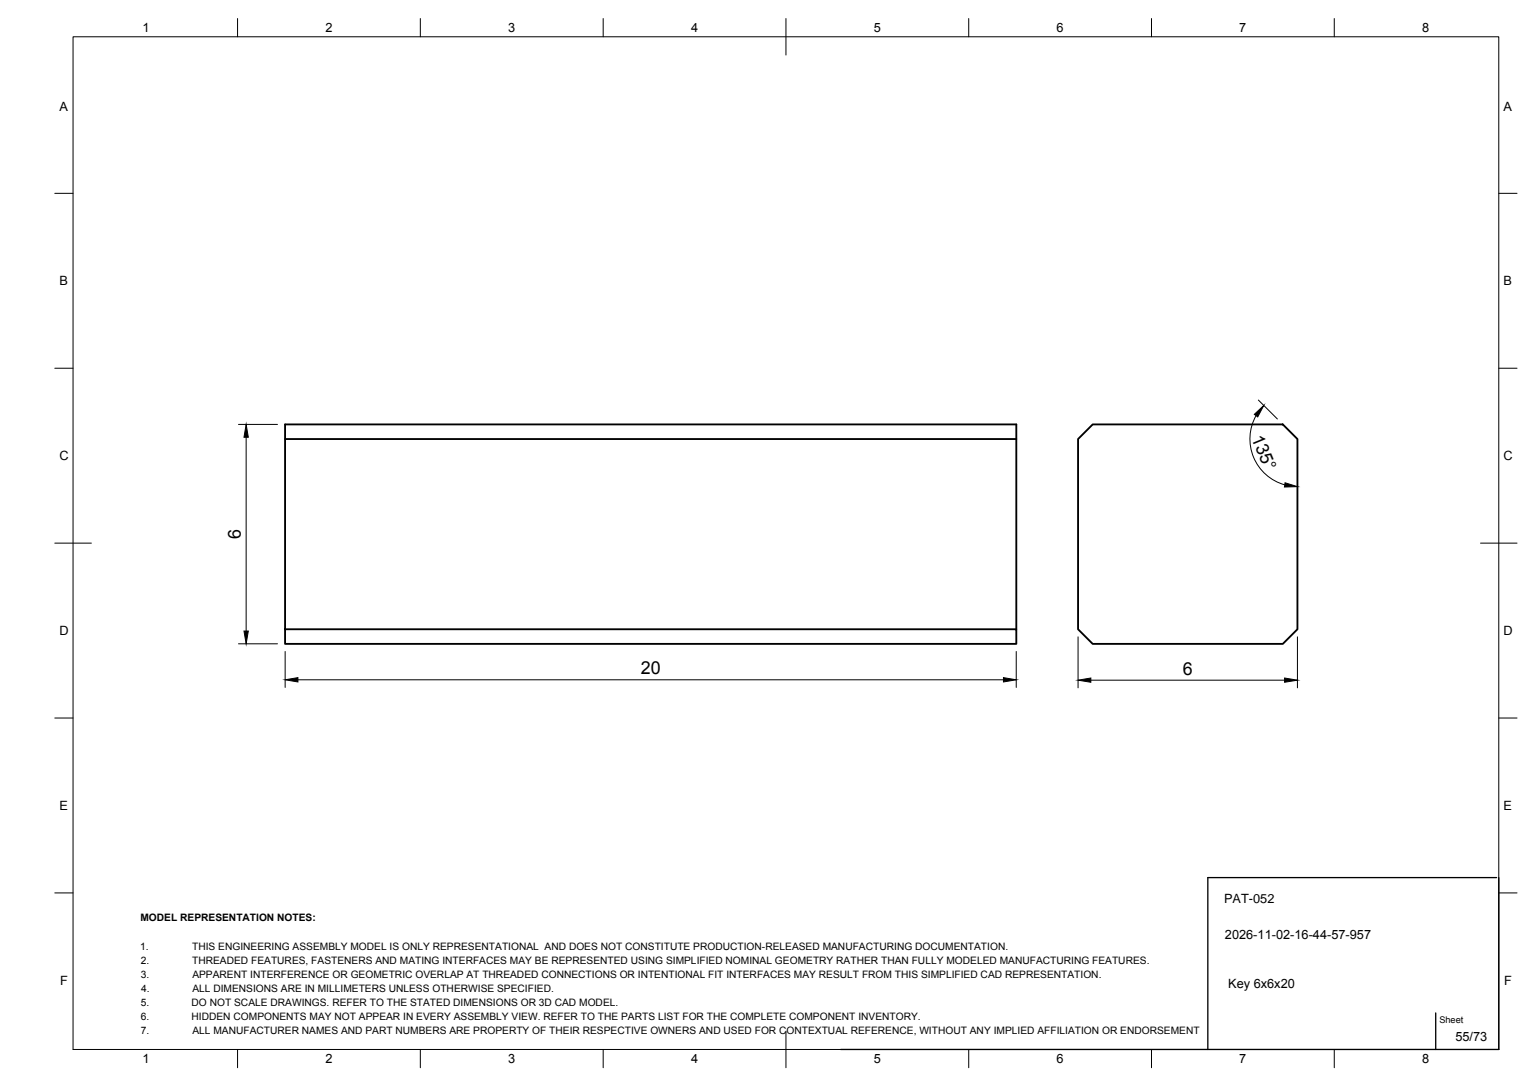
ISO-10303-21;
HEADER;
/* Generated by software containing ST-Developer
 * from STEP Tools, Inc. (www.steptools.com) 
 */

FILE_DESCRIPTION(
/* description */ ('Hand-crank gear train demonstrator'),
/* implementation_level */ '2;1');

FILE_NAME(
/* name */ 'Key 6x6x20.step',
/* time_stamp */ '2026-10-28T03:22:13-07:00',
/* author */ (''),
/* organization */ (''),
/* preprocessor_version */ 'ST-DEVELOPER v20.2',
/* originating_system */ 'Autodesk Translation Framework v15.17.0.0',
/* authorisation */ '');

FILE_SCHEMA (('AUTOMOTIVE_DESIGN { 1 0 10303 214 3 1 1 }'));
ENDSEC;

DATA;
#10=MECHANICAL_DESIGN_GEOMETRIC_PRESENTATION_REPRESENTATION('',(#1264),#62758);
#1121=SHAPE_REPRESENTATION_RELATIONSHIP('SRR','None',#63099,#1185);
#1185=ADVANCED_BREP_SHAPE_REPRESENTATION('',(#1339),#62753);
#1264=STYLED_ITEM('',(#63462),#1339);
#1339=MANIFOLD_SOLID_BREP('Body1',#16448);
#2091=PLANE('',#18656);
#2092=PLANE('',#18657);
#2093=PLANE('',#18658);
#2094=PLANE('',#18659);
#2095=PLANE('',#18660);
#2096=PLANE('',#18661);
#2097=PLANE('',#18662);
#2098=PLANE('',#18663);
#2099=PLANE('',#18664);
#2100=PLANE('',#18665);
#3016=FACE_OUTER_BOUND('',#4239,.T.);
#3017=FACE_OUTER_BOUND('',#4240,.T.);
#3018=FACE_OUTER_BOUND('',#4241,.T.);
#3019=FACE_OUTER_BOUND('',#4242,.T.);
#3020=FACE_OUTER_BOUND('',#4243,.T.);
#3021=FACE_OUTER_BOUND('',#4244,.T.);
#3022=FACE_OUTER_BOUND('',#4245,.T.);
#3023=FACE_OUTER_BOUND('',#4246,.T.);
#3024=FACE_OUTER_BOUND('',#4247,.T.);
#3025=FACE_OUTER_BOUND('',#4248,.T.);
#4239=EDGE_LOOP('',(#14993,#14994,#14995,#14996,#14997,#14998,#14999,#15000));
#4240=EDGE_LOOP('',(#15001,#15002,#15003,#15004));
#4241=EDGE_LOOP('',(#15005,#15006,#15007,#15008));
#4242=EDGE_LOOP('',(#15009,#15010,#15011,#15012));
#4243=EDGE_LOOP('',(#15013,#15014,#15015,#15016));
#4244=EDGE_LOOP('',(#15017,#15018,#15019,#15020,#15021,#15022,#15023,#15024));
#4245=EDGE_LOOP('',(#15025,#15026,#15027,#15028));
#4246=EDGE_LOOP('',(#15029,#15030,#15031,#15032));
#4247=EDGE_LOOP('',(#15033,#15034,#15035,#15036));
#4248=EDGE_LOOP('',(#15037,#15038,#15039,#15040));
#5347=LINE('',#62312,#6479);
#5348=LINE('',#62314,#6480);
#5349=LINE('',#62316,#6481);
#5350=LINE('',#62318,#6482);
#5351=LINE('',#62320,#6483);
#5352=LINE('',#62322,#6484);
#5353=LINE('',#62324,#6485);
#5354=LINE('',#62325,#6486);
#5355=LINE('',#62328,#6487);
#5356=LINE('',#62330,#6488);
#5357=LINE('',#62331,#6489);
#5358=LINE('',#62334,#6490);
#5359=LINE('',#62335,#6491);
#5360=LINE('',#62338,#6492);
#5361=LINE('',#62339,#6493);
#5362=LINE('',#62342,#6494);
#5363=LINE('',#62343,#6495);
#5364=LINE('',#62347,#6496);
#5365=LINE('',#62348,#6497);
#5366=LINE('',#62350,#6498);
#5367=LINE('',#62351,#6499);
#5368=LINE('',#62353,#6500);
#5369=LINE('',#62355,#6501);
#5370=LINE('',#62357,#6502);
#6479=VECTOR('',#22890,1.);
#6480=VECTOR('',#22891,1.);
#6481=VECTOR('',#22892,1.);
#6482=VECTOR('',#22893,1.);
#6483=VECTOR('',#22894,1.);
#6484=VECTOR('',#22895,1.);
#6485=VECTOR('',#22896,1.);
#6486=VECTOR('',#22897,1.);
#6487=VECTOR('',#22900,1.);
#6488=VECTOR('',#22901,1.);
#6489=VECTOR('',#22902,1.);
#6490=VECTOR('',#22905,1.);
#6491=VECTOR('',#22906,1.);
#6492=VECTOR('',#22909,1.);
#6493=VECTOR('',#22910,1.);
#6494=VECTOR('',#22913,1.);
#6495=VECTOR('',#22914,1.);
#6496=VECTOR('',#22917,1.);
#6497=VECTOR('',#22918,1.);
#6498=VECTOR('',#22919,1.);
#6499=VECTOR('',#22920,1.);
#6500=VECTOR('',#22923,1.);
#6501=VECTOR('',#22926,1.);
#6502=VECTOR('',#22929,1.);
#8613=VERTEX_POINT('',#62310);
#8614=VERTEX_POINT('',#62311);
#8615=VERTEX_POINT('',#62313);
#8616=VERTEX_POINT('',#62315);
#8617=VERTEX_POINT('',#62317);
#8618=VERTEX_POINT('',#62319);
#8619=VERTEX_POINT('',#62321);
#8620=VERTEX_POINT('',#62323);
#8621=VERTEX_POINT('',#62327);
#8622=VERTEX_POINT('',#62329);
#8623=VERTEX_POINT('',#62333);
#8624=VERTEX_POINT('',#62337);
#8625=VERTEX_POINT('',#62341);
#8626=VERTEX_POINT('',#62345);
#8627=VERTEX_POINT('',#62346);
#8628=VERTEX_POINT('',#62349);
#10748=EDGE_CURVE('',#8613,#8614,#5347,.T.);
#10749=EDGE_CURVE('',#8615,#8613,#5348,.T.);
#10750=EDGE_CURVE('',#8616,#8615,#5349,.T.);
#10751=EDGE_CURVE('',#8617,#8616,#5350,.T.);
#10752=EDGE_CURVE('',#8618,#8617,#5351,.T.);
#10753=EDGE_CURVE('',#8619,#8618,#5352,.T.);
#10754=EDGE_CURVE('',#8620,#8619,#5353,.T.);
#10755=EDGE_CURVE('',#8614,#8620,#5354,.T.);
#10756=EDGE_CURVE('',#8617,#8621,#5355,.T.);
#10757=EDGE_CURVE('',#8621,#8622,#5356,.T.);
#10758=EDGE_CURVE('',#8622,#8618,#5357,.T.);
#10759=EDGE_CURVE('',#8623,#8616,#5358,.T.);
#10760=EDGE_CURVE('',#8623,#8621,#5359,.T.);
#10761=EDGE_CURVE('',#8615,#8624,#5360,.T.);
#10762=EDGE_CURVE('',#8624,#8623,#5361,.T.);
#10763=EDGE_CURVE('',#8625,#8613,#5362,.T.);
#10764=EDGE_CURVE('',#8625,#8624,#5363,.T.);
#10765=EDGE_CURVE('',#8626,#8627,#5364,.T.);
#10766=EDGE_CURVE('',#8622,#8626,#5365,.T.);
#10767=EDGE_CURVE('',#8628,#8625,#5366,.T.);
#10768=EDGE_CURVE('',#8627,#8628,#5367,.T.);
#10769=EDGE_CURVE('',#8619,#8626,#5368,.T.);
#10770=EDGE_CURVE('',#8614,#8628,#5369,.T.);
#10771=EDGE_CURVE('',#8627,#8620,#5370,.T.);
#14993=ORIENTED_EDGE('',*,*,#10748,.F.);
#14994=ORIENTED_EDGE('',*,*,#10749,.F.);
#14995=ORIENTED_EDGE('',*,*,#10750,.F.);
#14996=ORIENTED_EDGE('',*,*,#10751,.F.);
#14997=ORIENTED_EDGE('',*,*,#10752,.F.);
#14998=ORIENTED_EDGE('',*,*,#10753,.F.);
#14999=ORIENTED_EDGE('',*,*,#10754,.F.);
#15000=ORIENTED_EDGE('',*,*,#10755,.F.);
#15001=ORIENTED_EDGE('',*,*,#10752,.T.);
#15002=ORIENTED_EDGE('',*,*,#10756,.T.);
#15003=ORIENTED_EDGE('',*,*,#10757,.T.);
#15004=ORIENTED_EDGE('',*,*,#10758,.T.);
#15005=ORIENTED_EDGE('',*,*,#10751,.T.);
#15006=ORIENTED_EDGE('',*,*,#10759,.F.);
#15007=ORIENTED_EDGE('',*,*,#10760,.T.);
#15008=ORIENTED_EDGE('',*,*,#10756,.F.);
#15009=ORIENTED_EDGE('',*,*,#10750,.T.);
#15010=ORIENTED_EDGE('',*,*,#10761,.T.);
#15011=ORIENTED_EDGE('',*,*,#10762,.T.);
#15012=ORIENTED_EDGE('',*,*,#10759,.T.);
#15013=ORIENTED_EDGE('',*,*,#10749,.T.);
#15014=ORIENTED_EDGE('',*,*,#10763,.F.);
#15015=ORIENTED_EDGE('',*,*,#10764,.T.);
#15016=ORIENTED_EDGE('',*,*,#10761,.F.);
#15017=ORIENTED_EDGE('',*,*,#10765,.F.);
#15018=ORIENTED_EDGE('',*,*,#10766,.F.);
#15019=ORIENTED_EDGE('',*,*,#10757,.F.);
#15020=ORIENTED_EDGE('',*,*,#10760,.F.);
#15021=ORIENTED_EDGE('',*,*,#10762,.F.);
#15022=ORIENTED_EDGE('',*,*,#10764,.F.);
#15023=ORIENTED_EDGE('',*,*,#10767,.F.);
#15024=ORIENTED_EDGE('',*,*,#10768,.F.);
#15025=ORIENTED_EDGE('',*,*,#10753,.T.);
#15026=ORIENTED_EDGE('',*,*,#10758,.F.);
#15027=ORIENTED_EDGE('',*,*,#10766,.T.);
#15028=ORIENTED_EDGE('',*,*,#10769,.F.);
#15029=ORIENTED_EDGE('',*,*,#10748,.T.);
#15030=ORIENTED_EDGE('',*,*,#10770,.T.);
#15031=ORIENTED_EDGE('',*,*,#10767,.T.);
#15032=ORIENTED_EDGE('',*,*,#10763,.T.);
#15033=ORIENTED_EDGE('',*,*,#10754,.T.);
#15034=ORIENTED_EDGE('',*,*,#10769,.T.);
#15035=ORIENTED_EDGE('',*,*,#10765,.T.);
#15036=ORIENTED_EDGE('',*,*,#10771,.T.);
#15037=ORIENTED_EDGE('',*,*,#10755,.T.);
#15038=ORIENTED_EDGE('',*,*,#10771,.F.);
#15039=ORIENTED_EDGE('',*,*,#10768,.T.);
#15040=ORIENTED_EDGE('',*,*,#10770,.F.);
#16326=ADVANCED_FACE('',(#3016),#2091,.F.);
#16327=ADVANCED_FACE('',(#3017),#2092,.T.);
#16328=ADVANCED_FACE('',(#3018),#2093,.T.);
#16329=ADVANCED_FACE('',(#3019),#2094,.T.);
#16330=ADVANCED_FACE('',(#3020),#2095,.T.);
#16331=ADVANCED_FACE('',(#3021),#2096,.T.);
#16332=ADVANCED_FACE('',(#3022),#2097,.F.);
#16333=ADVANCED_FACE('',(#3023),#2098,.T.);
#16334=ADVANCED_FACE('',(#3024),#2099,.T.);
#16335=ADVANCED_FACE('',(#3025),#2100,.T.);
#16448=CLOSED_SHELL('',(#16326,#16327,#16328,#16329,#16330,#16331,#16332,
#16333,#16334,#16335));
#18655=AXIS2_PLACEMENT_3D('',#62308,#22886,#22887);
#18656=AXIS2_PLACEMENT_3D('',#62309,#22888,#22889);
#18657=AXIS2_PLACEMENT_3D('',#62326,#22898,#22899);
#18658=AXIS2_PLACEMENT_3D('',#62332,#22903,#22904);
#18659=AXIS2_PLACEMENT_3D('',#62336,#22907,#22908);
#18660=AXIS2_PLACEMENT_3D('',#62340,#22911,#22912);
#18661=AXIS2_PLACEMENT_3D('',#62344,#22915,#22916);
#18662=AXIS2_PLACEMENT_3D('',#62352,#22921,#22922);
#18663=AXIS2_PLACEMENT_3D('',#62354,#22924,#22925);
#18664=AXIS2_PLACEMENT_3D('',#62356,#22927,#22928);
#18665=AXIS2_PLACEMENT_3D('',#62358,#22930,#22931);
#22886=DIRECTION('axis',(0.,0.,1.));
#22887=DIRECTION('refdir',(1.,0.,0.));
#22888=DIRECTION('center_axis',(1.,0.,0.));
#22889=DIRECTION('ref_axis',(0.,0.,-1.));
#22890=DIRECTION('',(0.,-0.707106781186547,-0.707106781186548));
#22891=DIRECTION('',(0.,-1.,0.));
#22892=DIRECTION('',(0.,-0.707106781186547,0.707106781186548));
#22893=DIRECTION('',(0.,0.,1.));
#22894=DIRECTION('',(0.,0.707106781186547,0.707106781186548));
#22895=DIRECTION('',(0.,1.,0.));
#22896=DIRECTION('',(0.,0.707106781186547,-0.707106781186548));
#22897=DIRECTION('',(0.,0.,-1.));
#22898=DIRECTION('center_axis',(0.,0.707106781186548,-0.707106781186547));
#22899=DIRECTION('ref_axis',(-1.,0.,0.));
#22900=DIRECTION('',(1.,0.,0.));
#22901=DIRECTION('',(0.,-0.707106781186547,-0.707106781186548));
#22902=DIRECTION('',(-1.,0.,0.));
#22903=DIRECTION('center_axis',(0.,1.,0.));
#22904=DIRECTION('ref_axis',(-1.,0.,0.));
#22905=DIRECTION('',(-1.,0.,0.));
#22906=DIRECTION('',(0.,0.,-1.));
#22907=DIRECTION('center_axis',(0.,0.707106781186548,0.707106781186547));
#22908=DIRECTION('ref_axis',(1.,0.,0.));
#22909=DIRECTION('',(1.,0.,0.));
#22910=DIRECTION('',(0.,0.707106781186547,-0.707106781186548));
#22911=DIRECTION('center_axis',(0.,0.,1.));
#22912=DIRECTION('ref_axis',(1.,0.,0.));
#22913=DIRECTION('',(-1.,0.,0.));
#22914=DIRECTION('',(0.,1.,0.));
#22915=DIRECTION('center_axis',(1.,0.,0.));
#22916=DIRECTION('ref_axis',(0.,0.,-1.));
#22917=DIRECTION('',(0.,-0.707106781186547,0.707106781186548));
#22918=DIRECTION('',(0.,-1.,0.));
#22919=DIRECTION('',(0.,0.707106781186547,0.707106781186548));
#22920=DIRECTION('',(0.,0.,1.));
#22921=DIRECTION('center_axis',(0.,0.,1.));
#22922=DIRECTION('ref_axis',(1.,0.,0.));
#22923=DIRECTION('',(1.,0.,0.));
#22924=DIRECTION('center_axis',(0.,-0.707106781186548,0.707106781186547));
#22925=DIRECTION('ref_axis',(1.,0.,0.));
#22926=DIRECTION('',(1.,0.,0.));
#22927=DIRECTION('center_axis',(0.,-0.707106781186548,-0.707106781186547));
#22928=DIRECTION('ref_axis',(-1.,0.,0.));
#22929=DIRECTION('',(-1.,0.,0.));
#22930=DIRECTION('center_axis',(0.,-1.,0.));
#22931=DIRECTION('ref_axis',(1.,0.,0.));
#62308=CARTESIAN_POINT('',(0.,0.,0.));
#62309=CARTESIAN_POINT('Origin',(-1.,0.,0.35));
#62310=CARTESIAN_POINT('',(-1.,-0.26,0.6));
#62311=CARTESIAN_POINT('',(-1.,-0.3,0.56));
#62312=CARTESIAN_POINT('',(-1.,-0.2675,0.5925));
#62313=CARTESIAN_POINT('',(-1.,0.26,0.6));
#62314=CARTESIAN_POINT('',(-1.,0.,0.6));
#62315=CARTESIAN_POINT('',(-1.,0.3,0.56));
#62316=CARTESIAN_POINT('',(-1.,0.2675,0.5925));
#62317=CARTESIAN_POINT('',(-1.,0.3,0.04));
#62318=CARTESIAN_POINT('',(-1.,0.3,0.175));
#62319=CARTESIAN_POINT('',(-1.,0.26,0.));
#62320=CARTESIAN_POINT('',(-1.,0.2925,0.0325));
#62321=CARTESIAN_POINT('',(-1.,-0.26,0.));
#62322=CARTESIAN_POINT('',(-1.,0.,0.));
#62323=CARTESIAN_POINT('',(-1.,-0.3,0.04));
#62324=CARTESIAN_POINT('',(-1.,-0.2925,0.0325));
#62325=CARTESIAN_POINT('',(-1.,-0.3,0.175));
#62326=CARTESIAN_POINT('Origin',(0.75,0.28,0.02));
#62327=CARTESIAN_POINT('',(1.,0.3,0.04));
#62328=CARTESIAN_POINT('',(0.75,0.3,0.04));
#62329=CARTESIAN_POINT('',(1.,0.26,0.));
#62330=CARTESIAN_POINT('',(1.,0.2925,0.0325));
#62331=CARTESIAN_POINT('',(0.75,0.26,0.));
#62332=CARTESIAN_POINT('Origin',(1.5,0.3,0.));
#62333=CARTESIAN_POINT('',(1.,0.3,0.56));
#62334=CARTESIAN_POINT('',(0.75,0.3,0.56));
#62335=CARTESIAN_POINT('',(1.,0.3,0.175));
#62336=CARTESIAN_POINT('Origin',(0.75,0.28,0.58));
#62337=CARTESIAN_POINT('',(1.,0.26,0.6));
#62338=CARTESIAN_POINT('',(0.75,0.26,0.6));
#62339=CARTESIAN_POINT('',(1.,0.2675,0.5925));
#62340=CARTESIAN_POINT('Origin',(0.,0.,0.6));
#62341=CARTESIAN_POINT('',(1.,-0.26,0.6));
#62342=CARTESIAN_POINT('',(-0.75,-0.26,0.6));
#62343=CARTESIAN_POINT('',(1.,0.,0.6));
#62344=CARTESIAN_POINT('Origin',(1.,0.,0.35));
#62345=CARTESIAN_POINT('',(1.,-0.26,0.));
#62346=CARTESIAN_POINT('',(1.,-0.3,0.04));
#62347=CARTESIAN_POINT('',(1.,-0.2925,0.0325));
#62348=CARTESIAN_POINT('',(1.,0.,0.));
#62349=CARTESIAN_POINT('',(1.,-0.3,0.56));
#62350=CARTESIAN_POINT('',(1.,-0.2675,0.5925));
#62351=CARTESIAN_POINT('',(1.,-0.3,0.175));
#62352=CARTESIAN_POINT('Origin',(0.,0.,0.));
#62353=CARTESIAN_POINT('',(-0.75,-0.26,0.));
#62354=CARTESIAN_POINT('Origin',(-0.75,-0.28,0.58));
#62355=CARTESIAN_POINT('',(-0.75,-0.3,0.56));
#62356=CARTESIAN_POINT('Origin',(-0.75,-0.28,0.02));
#62357=CARTESIAN_POINT('',(-0.75,-0.3,0.04));
#62358=CARTESIAN_POINT('Origin',(-1.5,-0.3,0.));
#62679=UNCERTAINTY_MEASURE_WITH_UNIT(LENGTH_MEASURE(0.001),#62759,
'DISTANCE_ACCURACY_VALUE',
'Maximum model space distance between geometric entities at asserted c
onnectivities');
#62684=UNCERTAINTY_MEASURE_WITH_UNIT(LENGTH_MEASURE(0.001),#62759,
'DISTANCE_ACCURACY_VALUE',
'Maximum model space distance between geometric entities at asserted c
onnectivities');
#62753=(
GEOMETRIC_REPRESENTATION_CONTEXT(3)
GLOBAL_UNCERTAINTY_ASSIGNED_CONTEXT((#62679))
GLOBAL_UNIT_ASSIGNED_CONTEXT((#62759,#62761,#62762))
REPRESENTATION_CONTEXT('','3D')
);
#62758=(
GEOMETRIC_REPRESENTATION_CONTEXT(3)
GLOBAL_UNCERTAINTY_ASSIGNED_CONTEXT((#62684))
GLOBAL_UNIT_ASSIGNED_CONTEXT((#62759,#62761,#62762))
REPRESENTATION_CONTEXT('','3D')
);
#62759=(
LENGTH_UNIT()
NAMED_UNIT(*)
SI_UNIT(.CENTI.,.METRE.)
);
#62761=(
NAMED_UNIT(*)
PLANE_ANGLE_UNIT()
SI_UNIT($,.RADIAN.)
);
#62762=(
NAMED_UNIT(*)
SI_UNIT($,.STERADIAN.)
SOLID_ANGLE_UNIT()
);
#62831=SHAPE_DEFINITION_REPRESENTATION(#62914,#63099);
#62914=PRODUCT_DEFINITION_SHAPE('',$,#63173);
#63099=SHAPE_REPRESENTATION('',(#18655),#62753);
#63104=PRODUCT_DEFINITION_CONTEXT('part definition',#63325,'design');
#63173=PRODUCT_DEFINITION('Key 6x6x20','Key 6x6x20',#63246,#63104);
#63246=PRODUCT_DEFINITION_FORMATION('',$,#63395);
#63325=APPLICATION_CONTEXT(
'Core Data for Automotive Mechanical Design Process');
#63326=PRODUCT_CONTEXT('part definition',#63325,'mechanical');
#63395=PRODUCT('Key 6x6x20','Key 6x6x20','Key 6x6x20',(#63326));
#63456=COLOUR_RGB('Grey',0.48,0.52,0.57);
#63457=FILL_AREA_STYLE_COLOUR('',#63456);
#63458=FILL_AREA_STYLE('',(#63457));
#63459=SURFACE_STYLE_FILL_AREA(#63458);
#63460=SURFACE_SIDE_STYLE('',(#63459));
#63461=SURFACE_STYLE_USAGE(.BOTH.,#63460);
#63462=PRESENTATION_STYLE_ASSIGNMENT((#63461));
ENDSEC;
END-ISO-10303-21;
